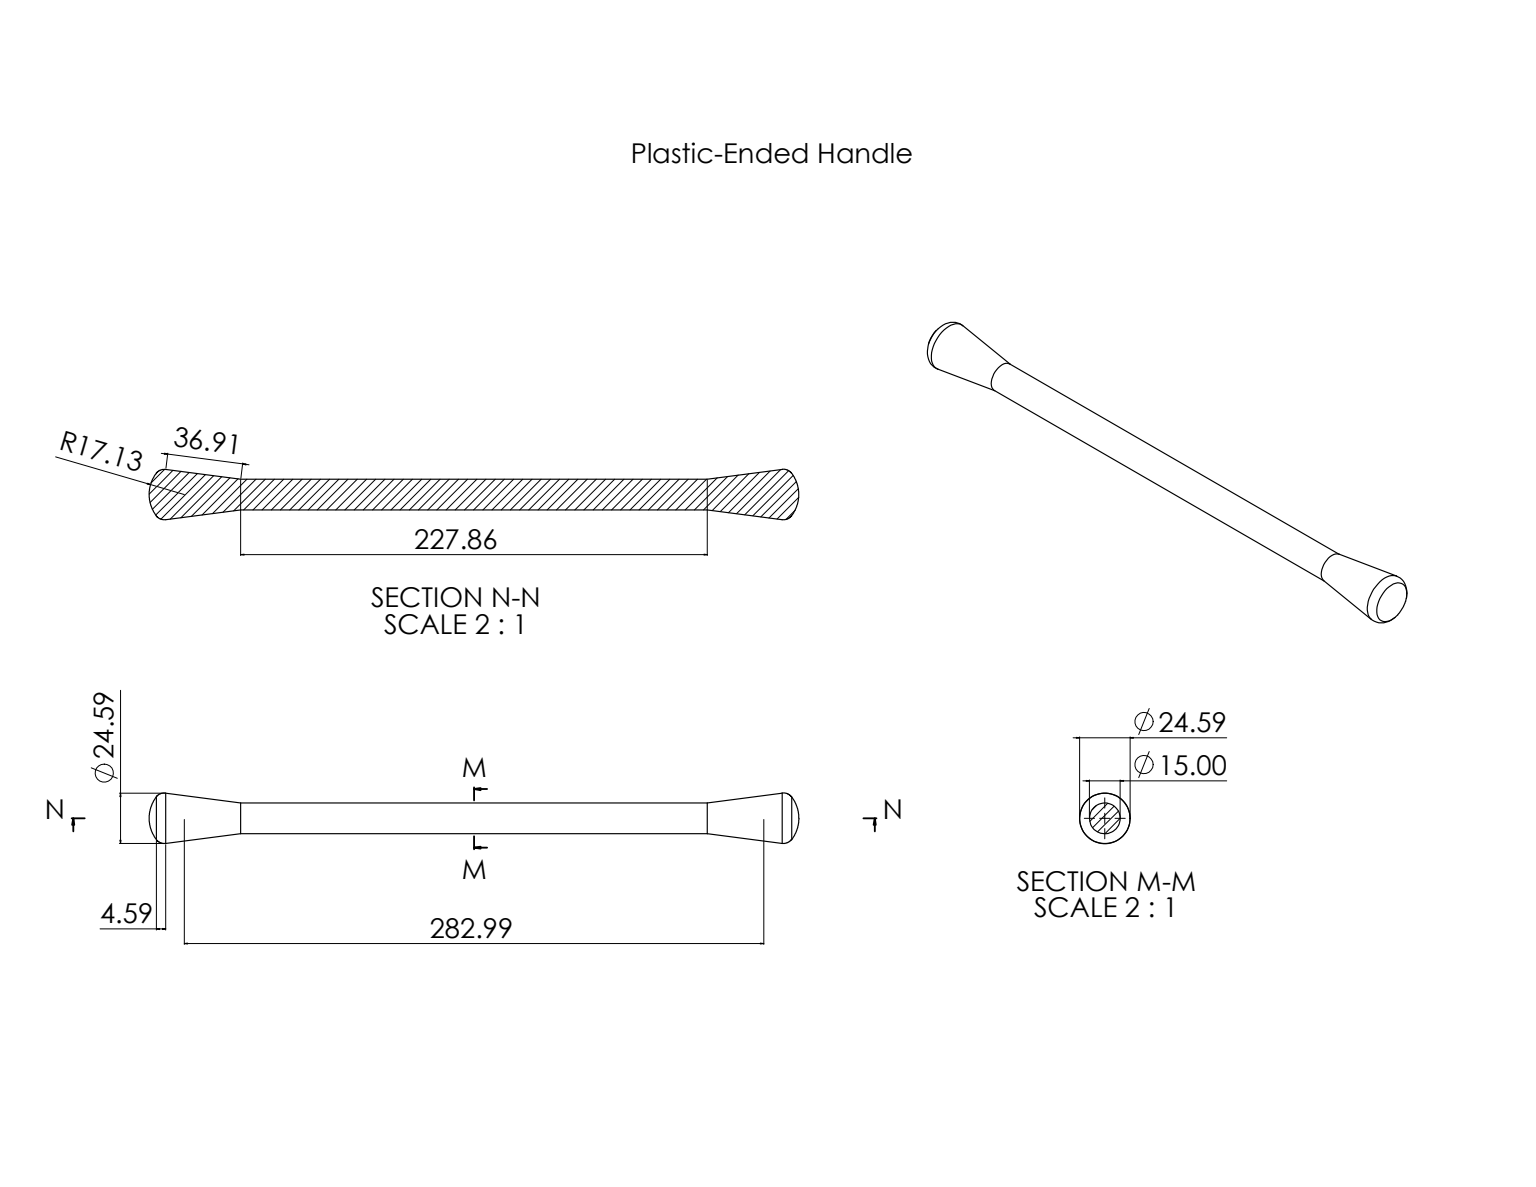
ISO-10303-21;
HEADER;
FILE_DESCRIPTION (('STEP AP214'),
    '1' );
FILE_NAME ('Plastic-Ended Handle.step',
    '2026-10-21T18:33:49',
    ( '' ),
    ( '' ),
    'SwSTEP 2.0',
    'SolidWorks 2025',
    '' );
FILE_SCHEMA (( 'AUTOMOTIVE_DESIGN' ));
ENDSEC;

DATA;
#11=AXIS2_PLACEMENT_3D ( 'NONE', #13563, #6445, #16272 ) ;
#14=ORIENTED_EDGE ( 'NONE', *, *, #12006, .F. ) ;
#41=LINE ( 'NONE', #15673, #2725 ) ;
#85=( NAMED_UNIT ( * ) SI_UNIT ( $, .STERADIAN. ) SOLID_ANGLE_UNIT ( ) );
#126=ADVANCED_FACE ( 'NONE', ( #11640 ), #16856, .T. ) ;
#152=MANIFOLD_SOLID_BREP ( 'Revolve1', #15042 ) ;
#157=CIRCLE ( 'NONE', #3134, 10.38004356723770627 ) ;
#223=DIRECTION ( 'NONE',  ( 0.000000000000000000, -0.000000000000000000, 1.000000000000000000 ) ) ;
#307=CIRCLE ( 'NONE', #13165, 4.962965561209093046 ) ;
#345=ORIENTED_EDGE ( 'NONE', *, *, #13737, .F. ) ;
#374=CARTESIAN_POINT ( 'NONE',  ( -212.2032458117903104, 84.22855780814606419, 52.11995643276230794 ) ) ;
#389=DIRECTION ( 'NONE',  ( 0.000000000000000000, 0.000000000000000000, 1.000000000000000000 ) ) ;
#392=ORIENTED_EDGE ( 'NONE', *, *, #13744, .T. ) ;
#655=AXIS2_PLACEMENT_3D ( 'NONE', #13524, #709, #7704 ) ;
#658=ORIENTED_EDGE ( 'NONE', *, *, #15578, .F. ) ;
#681=CARTESIAN_POINT ( 'NONE',  ( -208.2552686774341737, 84.22855780814606419, 55.12736457073573604 ) ) ;
#709=DIRECTION ( 'NONE',  ( 0.000000000000000000, -0.000000000000000000, -1.000000000000000000 ) ) ;
#801=LINE ( 'NONE', #2012, #10914 ) ;
#819=DIRECTION ( 'NONE',  ( 0.000000000000000000, 0.000000000000000000, -1.000000000000000000 ) ) ;
#822=EDGE_CURVE ( 'NONE', #1101, #833, #157, .T. ) ;
#833=VERTEX_POINT ( 'NONE', #374 ) ;
#864=VERTEX_POINT ( 'NONE', #11793 ) ;
#905=FACE_OUTER_BOUND ( 'NONE', #13588, .T. ) ;
#932=CARTESIAN_POINT ( 'NONE',  ( -171.0109138863553824, 84.22855780814606419, 55.00000000000000711 ) ) ;
#942=DIRECTION ( 'NONE',  ( 1.000000000000000000, -0.000000000000000000, -0.000000000000000000 ) ) ;
#992=DIRECTION ( 'NONE',  ( 0.000000000000000000, 0.000000000000000000, 1.000000000000000000 ) ) ;
#998=ORIENTED_EDGE ( 'NONE', *, *, #15679, .F. ) ;
#1033=DIRECTION ( 'NONE',  ( -0.9915318908039647550, 1.590368294782254281E-17, -0.1298634264091108326 ) ) ;
#1101=VERTEX_POINT ( 'NONE', #4112 ) ;
#1111=FACE_OUTER_BOUND ( 'NONE', #17441, .T. ) ;
#1270=ORIENTED_EDGE ( 'NONE', *, *, #2418, .T. ) ;
#1305=FACE_OUTER_BOUND ( 'NONE', #5820, .T. ) ;
#1431=EDGE_LOOP ( 'NONE', ( #9618, #16149, #15476, #8955 ) ) ;
#1443=ORIENTED_EDGE ( 'NONE', *, *, #5918, .F. ) ;
#1466=CARTESIAN_POINT ( 'NONE',  ( 93.45071565215914688, 84.22855780814606419, 62.50000000000001421 ) ) ;
#1568=ORIENTED_EDGE ( 'NONE', *, *, #6498, .F. ) ;
#1660=FACE_OUTER_BOUND ( 'NONE', #4429, .T. ) ;
#1677=SHAPE_REPRESENTATION ( 'Plastic-Ended Handle', ( #16217 ), #12057 ) ;
#1703=CARTESIAN_POINT ( 'NONE',  ( -212.2032458117903104, 84.22855780814606419, 72.88004356723772048 ) ) ;
#1752=CARTESIAN_POINT ( 'NONE',  ( 93.45071565215914688, 84.22855780814606419, 74.79357405616491405 ) ) ;
#1784=DIRECTION ( 'NONE',  ( -1.000000000000000000, -0.000000000000000000, -0.000000000000000000 ) ) ;
#1810=ADVANCED_FACE ( 'NONE', ( #905 ), #6119, .T. ) ;
#1833=AXIS2_PLACEMENT_3D ( 'NONE', #11522, #4305, #10972 ) ;
#1834=ADVANCED_FACE ( 'NONE', ( #1111 ), #9012, .T. ) ;
#1908=VERTEX_POINT ( 'NONE', #9897 ) ;
#2012=CARTESIAN_POINT ( 'NONE',  ( 97.91997734382704266, 84.22855780814606419, 70.00000000000001421 ) ) ;
#2048=EDGE_CURVE ( 'NONE', #833, #4354, #17752, .T. ) ;
#2060=FACE_OUTER_BOUND ( 'NONE', #8644, .T. ) ;
#2093=( NAMED_UNIT ( * ) SI_UNIT ( $, .STERADIAN. ) SOLID_ANGLE_UNIT ( ) );
#2118=LINE ( 'NONE', #15207, #8794 ) ;
#2381=CIRCLE ( 'NONE', #12873, 17.12963335357822814 ) ;
#2418=EDGE_CURVE ( 'NONE', #10909, #17887, #10092, .T. ) ;
#2423=LINE ( 'NONE', #932, #15542 ) ;
#2440=AXIS2_PLACEMENT_3D ( 'NONE', #5540, #18168, #13966 ) ;
#2474=CIRCLE ( 'NONE', #3078, 10.38004356723770627 ) ;
#2503=APPLICATION_CONTEXT ( 'automotive_design' ) ;
#2540=MECHANICAL_DESIGN_GEOMETRIC_PRESENTATION_REPRESENTATION('',(#6710),#15684);
#2587=CARTESIAN_POINT ( 'NONE',  ( 97.91997734382704266, 84.22855780814606419, 62.50000000000001421 ) ) ;
#2663=ADVANCED_FACE ( 'NONE', ( #6795 ), #13556, .T. ) ;
#2674=DIRECTION ( 'NONE',  ( 1.000000000000000000, -0.000000000000000000, -0.000000000000000000 ) ) ;
#2679=PRODUCT ( 'Plastic-Ended Handle', 'Plastic-Ended Handle', '', ( #6865 ) ) ;
#2725=VECTOR ( 'NONE', #8469, 1000.000000000000000 ) ;
#2771=CARTESIAN_POINT ( 'NONE',  ( 84.41679105416972106, 84.22855780814606419, 62.50000000000001421 ) ) ;
#2872=AXIS2_PLACEMENT_3D ( 'NONE', #13058, #223, #8747 ) ;
#2969=CARTESIAN_POINT ( 'NONE',  ( 93.45071565215914688, 84.22855780814606419, 62.50000000000001421 ) ) ;
#3004=DIRECTION ( 'NONE',  ( 1.000000000000000000, -0.000000000000000000, -0.000000000000000000 ) ) ;
#3050=VERTEX_POINT ( 'NONE', #1703 ) ;
#3078=AXIS2_PLACEMENT_3D ( 'NONE', #6362, #9279, #12180 ) ;
#3122=AXIS2_PLACEMENT_3D ( 'NONE', #7521, #10240, #8854 ) ;
#3134=AXIS2_PLACEMENT_3D ( 'NONE', #4485, #3004, #15904 ) ;
#3167=VERTEX_POINT ( 'NONE', #6171 ) ;
#3255=ORIENTED_EDGE ( 'NONE', *, *, #15679, .T. ) ;
#3357=DIRECTION ( 'NONE',  ( -1.000000000000000000, 0.000000000000000000, 0.000000000000000000 ) ) ;
#3455=ORIENTED_EDGE ( 'NONE', *, *, #9148, .T. ) ;
#3495=DIRECTION ( 'NONE',  ( 1.000000000000000000, -0.000000000000000000, -0.000000000000000000 ) ) ;
#3565=DIRECTION ( 'NONE',  ( 0.000000000000000000, 1.000000000000000000, 0.000000000000000000 ) ) ;
#3837=AXIS2_PLACEMENT_3D ( 'NONE', #3931, #5242, #9543 ) ;
#3850=DIRECTION ( 'NONE',  ( 0.000000000000000000, 0.000000000000000000, -1.000000000000000000 ) ) ;
#3862=( NAMED_UNIT ( * ) PLANE_ANGLE_UNIT ( ) SI_UNIT ( $, .RADIAN. ) );
#3931=CARTESIAN_POINT ( 'NONE',  ( 56.85086857400936822, 84.22855780814606419, 62.50000000000001421 ) ) ;
#3950=DIRECTION ( 'NONE',  ( 0.000000000000000000, 1.000000000000000000, 0.000000000000000000 ) ) ;
#4112=CARTESIAN_POINT ( 'NONE',  ( -212.2032458117903104, 73.84851424090838634, 62.50000000000001421 ) ) ;
#4252=DIRECTION ( 'NONE',  ( 0.000000000000000000, 0.000000000000000000, -1.000000000000000000 ) ) ;
#4305=DIRECTION ( 'NONE',  ( 1.000000000000000000, -0.000000000000000000, -0.000000000000000000 ) ) ;
#4354=VERTEX_POINT ( 'NONE', #16482 ) ;
#4429=EDGE_LOOP ( 'NONE', ( #18514, #18372, #3255, #18470 ) ) ;
#4449=EDGE_CURVE ( 'NONE', #864, #1101, #2381, .T. ) ;
#4485=CARTESIAN_POINT ( 'NONE',  ( -212.2032458117903104, 84.22855780814606419, 62.50000000000001421 ) ) ;
#4558=DIRECTION ( 'NONE',  ( 0.000000000000000000, 0.000000000000000000, -1.000000000000000000 ) ) ;
#4603=EDGE_CURVE ( 'NONE', #1908, #12880, #7466, .T. ) ;
#4635=AXIS2_PLACEMENT_3D ( 'NONE', #7678, #1784, #389 ) ;
#4769=ORIENTED_EDGE ( 'NONE', *, *, #822, .T. ) ;
#4877=DIRECTION ( 'NONE',  ( -0.9915318908039647550, 0.000000000000000000, 0.1298634264091108326 ) ) ;
#4894=CARTESIAN_POINT ( 'NONE',  ( -208.2552686774341737, 84.22855780814606419, 62.50000000000001421 ) ) ;
#4987=CARTESIAN_POINT ( 'NONE',  ( -212.2032458117903104, 84.22855780814606419, 62.50000000000001421 ) ) ;
#5020=EDGE_CURVE ( 'NONE', #17887, #12880, #307, .T. ) ;
#5087=ORIENTED_EDGE ( 'NONE', *, *, #6881, .T. ) ;
#5184=ORIENTED_EDGE ( 'NONE', *, *, #4449, .F. ) ;
#5223=ORIENTED_EDGE ( 'NONE', *, *, #8129, .T. ) ;
#5241=CIRCLE ( 'NONE', #18404, 10.38004356723770627 ) ;
#5242=DIRECTION ( 'NONE',  ( 1.000000000000000000, -0.000000000000000000, -0.000000000000000000 ) ) ;
#5280=EDGE_CURVE ( 'NONE', #14482, #14175, #17268, .T. ) ;
#5289=DIRECTION ( 'NONE',  ( 1.000000000000000000, 0.000000000000000000, 0.000000000000000000 ) ) ;
#5337=VERTEX_POINT ( 'NONE', #6377 ) ;
#5425=VERTEX_POINT ( 'NONE', #12004 ) ;
#5500=DIRECTION ( 'NONE',  ( 1.000000000000000000, -0.000000000000000000, -0.000000000000000000 ) ) ;
#5540=CARTESIAN_POINT ( 'NONE',  ( -207.6107609645051753, 84.22855780814606419, 62.50000000000001421 ) ) ;
#5575=ORIENTED_EDGE ( 'NONE', *, *, #7982, .T. ) ;
#5647=DIRECTION ( 'NONE',  ( 1.000000000000000000, -0.000000000000000000, -0.000000000000000000 ) ) ;
#5720=DIRECTION ( 'NONE',  ( 0.000000000000000000, 1.224646799147353207E-16, 1.000000000000000000 ) ) ;
#5750=CIRCLE ( 'NONE', #6638, 7.500000000000007105 ) ;
#5781=CARTESIAN_POINT ( 'NONE',  ( 0.000000000000000000, 0.000000000000000000, 0.000000000000000000 ) ) ;
#5800=CIRCLE ( 'NONE', #7899, 10.38004356723770627 ) ;
#5820=EDGE_LOOP ( 'NONE', ( #10610, #14671, #3455, #345 ) ) ;
#5883=CARTESIAN_POINT ( 'NONE',  ( 98.04320049944426785, 84.22855780814606419, 62.50000000000001421 ) ) ;
#5898=ADVANCED_BREP_SHAPE_REPRESENTATION ( '', ( #152, #16217 ), #12057 ) ;
#5918=EDGE_CURVE ( 'NONE', #10909, #5337, #12211, .T. ) ;
#6005=ORIENTED_EDGE ( 'NONE', *, *, #9042, .T. ) ;
#6011=CIRCLE ( 'NONE', #2440, 12.29357405616490695 ) ;
#6037=DIRECTION ( 'NONE',  ( 0.000000000000000000, 0.000000000000000000, 1.000000000000000000 ) ) ;
#6117=EDGE_CURVE ( 'NONE', #12880, #3167, #8386, .T. ) ;
#6119=CONICAL_SURFACE ( 'NONE', #16585, 12.29357405616490695, 0.1302312384721128480 ) ;
#6171=CARTESIAN_POINT ( 'NONE',  ( 98.04320049944426785, 94.60860137538374204, 62.50000000000001421 ) ) ;
#6215=( LENGTH_UNIT ( ) NAMED_UNIT ( * ) SI_UNIT ( .MILLI., .METRE. ) );
#6362=CARTESIAN_POINT ( 'NONE',  ( -212.2032458117903104, 84.22855780814606419, 62.50000000000001421 ) ) ;
#6377=CARTESIAN_POINT ( 'NONE',  ( 56.85086857400936822, 84.22855780814606419, 70.00000000000001421 ) ) ;
#6445=DIRECTION ( 'NONE',  ( 0.000000000000000000, 1.000000000000000000, -1.224646799147353207E-16 ) ) ;
#6498=EDGE_CURVE ( 'NONE', #5337, #11425, #41, .T. ) ;
#6559=DIRECTION ( 'NONE',  ( -0.000000000000000000, -1.000000000000000000, -0.000000000000000000 ) ) ;
#6579=DIRECTION ( 'NONE',  ( 1.000000000000000000, -0.000000000000000000, -0.000000000000000000 ) ) ;
#6620=ORIENTED_EDGE ( 'NONE', *, *, #5280, .T. ) ;
#6638=AXIS2_PLACEMENT_3D ( 'NONE', #15753, #11720, #15836 ) ;
#6652=UNCERTAINTY_MEASURE_WITH_UNIT (LENGTH_MEASURE( 1.000000000000000082E-05 ), #6215, 'distance_accuracy_value', 'NONE');
#6676=ORIENTED_EDGE ( 'NONE', *, *, #12311, .F. ) ;
#6692=DIRECTION ( 'NONE',  ( 0.000000000000000000, 0.000000000000000000, -1.000000000000000000 ) ) ;
#6710=STYLED_ITEM('',(#18545),#152);
#6795=FACE_OUTER_BOUND ( 'NONE', #10659, .T. ) ;
#6865=PRODUCT_CONTEXT ( 'NONE', #2503, 'mechanical' ) ;
#6881=EDGE_CURVE ( 'NONE', #11425, #17887, #14110, .T. ) ;
#6921=AXIS2_PLACEMENT_3D ( 'NONE', #18476, #5647, #4252 ) ;
#7039=FACE_OUTER_BOUND ( 'NONE', #11821, .T. ) ;
#7136=VERTEX_POINT ( 'NONE', #14683 ) ;
#7191=SHAPE_REPRESENTATION_RELATIONSHIP ( 'NONE' , 'NONE' ,  #1677, #5898 ) ;
#7208=CARTESIAN_POINT ( 'NONE',  ( 94.09522336508815954, 84.22855780814606419, 62.50000000000001421 ) ) ;
#7369=DIRECTION ( 'NONE',  ( 0.000000000000000000, -0.000000000000000000, -1.000000000000000000 ) ) ;
#7370=CARTESIAN_POINT ( 'NONE',  ( -171.0109138863553824, 84.22855780814606419, 62.50000000000001421 ) ) ;
#7387=DIRECTION ( 'NONE',  ( 0.000000000000000000, 0.000000000000000000, -1.000000000000000000 ) ) ;
#7420=EDGE_LOOP ( 'NONE', ( #17630, #16514, #6005, #16324 ) ) ;
#7466=CIRCLE ( 'NONE', #17907, 10.38004356723770627 ) ;
#7520=AXIS2_PLACEMENT_3D ( 'NONE', #13096, #9923, #11596 ) ;
#7521=CARTESIAN_POINT ( 'NONE',  ( -208.2552686774341737, 84.22855780814606419, 62.50000000000001421 ) ) ;
#7546=DIRECTION ( 'NONE',  ( 0.9915318908039647550, 0.000000000000000000, -0.1298634264091108326 ) ) ;
#7566=ADVANCED_FACE ( 'NONE', ( #7711 ), #14905, .T. ) ;
#7654=CARTESIAN_POINT ( 'NONE',  ( 94.09522336508815954, 84.22855780814606419, 55.12736457073573604 ) ) ;
#7662=ADVANCED_FACE ( 'NONE', ( #10699 ), #10517, .T. ) ;
#7678=CARTESIAN_POINT ( 'NONE',  ( 97.91997734382704266, 84.22855780814606419, 62.50000000000001421 ) ) ;
#7681=ORIENTED_EDGE ( 'NONE', *, *, #12311, .T. ) ;
#7704=DIRECTION ( 'NONE',  ( 0.000000000000000000, -1.000000000000000000, 0.000000000000000000 ) ) ;
#7711=FACE_OUTER_BOUND ( 'NONE', #1431, .T. ) ;
#7771=ORIENTED_EDGE ( 'NONE', *, *, #9729, .F. ) ;
#7776=CARTESIAN_POINT ( 'NONE',  ( 93.45071565215914688, 84.22855780814606419, 50.20642594383511437 ) ) ;
#7858=DIRECTION ( 'NONE',  ( 0.000000000000000000, 0.000000000000000000, -1.000000000000000000 ) ) ;
#7899=AXIS2_PLACEMENT_3D ( 'NONE', #4987, #6579, #10620 ) ;
#7982=EDGE_CURVE ( 'NONE', #5337, #10909, #5750, .T. ) ;
#8040=AXIS2_PLACEMENT_3D ( 'NONE', #7370, #13083, #10353 ) ;
#8054=DIRECTION ( 'NONE',  ( 1.000000000000000000, -0.000000000000000000, -0.000000000000000000 ) ) ;
#8064=CIRCLE ( 'NONE', #11, 4.962965561209093046 ) ;
#8129=EDGE_CURVE ( 'NONE', #10654, #3050, #2474, .T. ) ;
#8264=ORIENTED_EDGE ( 'NONE', *, *, #11575, .T. ) ;
#8310=ORIENTED_EDGE ( 'NONE', *, *, #6117, .F. ) ;
#8336=PRODUCT_DEFINITION_CONTEXT ( 'detailed design', #8853, 'design' ) ;
#8355=PRODUCT_DEFINITION_SHAPE ( 'NONE', 'NONE',  #15399 ) ;
#8386=CIRCLE ( 'NONE', #14361, 10.38004356723770627 ) ;
#8469=DIRECTION ( 'NONE',  ( 0.9915318908039647550, 1.590368294782254281E-17, 0.1298634264091108326 ) ) ;
#8472=EDGE_LOOP ( 'NONE', ( #5223, #16778, #998, #9687, #11073 ) ) ;
#8490=CARTESIAN_POINT ( 'NONE',  ( 56.85086857400936822, 84.22855780814606419, 55.00000000000000711 ) ) ;
#8493=PRODUCT_DEFINITION_FORMATION_WITH_SPECIFIED_SOURCE ( 'ANY', '', #2679, .NOT_KNOWN. ) ;
#8644=EDGE_LOOP ( 'NONE', ( #1443, #8264, #6620, #9226 ) ) ;
#8705=CARTESIAN_POINT ( 'NONE',  ( -171.0109138863553824, 84.22855780814606419, 70.00000000000001421 ) ) ;
#8747=DIRECTION ( 'NONE',  ( 0.000000000000000000, 1.000000000000000000, 0.000000000000000000 ) ) ;
#8794=VECTOR ( 'NONE', #15121, 1000.000000000000000 ) ;
#8853=APPLICATION_CONTEXT ( 'automotive_design' ) ;
#8854=DIRECTION ( 'NONE',  ( 0.000000000000000000, 0.000000000000000000, -1.000000000000000000 ) ) ;
#8904=CYLINDRICAL_SURFACE ( 'NONE', #4635, 7.500000000000007105 ) ;
#8953=EDGE_CURVE ( 'NONE', #833, #10654, #12905, .T. ) ;
#8955=ORIENTED_EDGE ( 'NONE', *, *, #13737, .T. ) ;
#8961=DIRECTION ( 'NONE',  ( 1.000000000000000000, 0.000000000000000000, 0.000000000000000000 ) ) ;
#8974=AXIS2_PLACEMENT_3D ( 'NONE', #10668, #16355, #9447 ) ;
#9012=SPHERICAL_SURFACE ( 'NONE', #2872, 17.12963335357822103 ) ;
#9042=EDGE_CURVE ( 'NONE', #14175, #7136, #16471, .T. ) ;
#9118=ORIENTED_EDGE ( 'NONE', *, *, #2418, .F. ) ;
#9148=EDGE_CURVE ( 'NONE', #3167, #5425, #17661, .T. ) ;
#9164=EDGE_CURVE ( 'NONE', #7136, #4354, #6011, .T. ) ;
#9226=ORIENTED_EDGE ( 'NONE', *, *, #13607, .F. ) ;
#9279=DIRECTION ( 'NONE',  ( 1.000000000000000000, -0.000000000000000000, -0.000000000000000000 ) ) ;
#9299=DIRECTION ( 'NONE',  ( 0.000000000000000000, 0.000000000000000000, -1.000000000000000000 ) ) ;
#9338=AXIS2_PLACEMENT_3D ( 'NONE', #4894, #3495, #9299 ) ;
#9360=CARTESIAN_POINT ( 'NONE',  ( 98.04320049944426785, 84.22855780814606419, 62.50000000000001421 ) ) ;
#9447=DIRECTION ( 'NONE',  ( 0.000000000000000000, 0.000000000000000000, -1.000000000000000000 ) ) ;
#9468=DIRECTION ( 'NONE',  ( 0.000000000000000000, 0.000000000000000000, -1.000000000000000000 ) ) ;
#9482=DIRECTION ( 'NONE',  ( 0.000000000000000000, 0.000000000000000000, 1.000000000000000000 ) ) ;
#9541=ORIENTED_EDGE ( 'NONE', *, *, #822, .F. ) ;
#9543=DIRECTION ( 'NONE',  ( 0.000000000000000000, 0.000000000000000000, -1.000000000000000000 ) ) ;
#9585=FACE_OUTER_BOUND ( 'NONE', #12427, .T. ) ;
#9618=ORIENTED_EDGE ( 'NONE', *, *, #9148, .F. ) ;
#9687=ORIENTED_EDGE ( 'NONE', *, *, #2048, .F. ) ;
#9729=EDGE_CURVE ( 'NONE', #3050, #7136, #13223, .T. ) ;
#9784=DIRECTION ( 'NONE',  ( 0.000000000000000000, 0.000000000000000000, 1.000000000000000000 ) ) ;
#9847=DIRECTION ( 'NONE',  ( 0.000000000000000000, -0.000000000000000000, 1.000000000000000000 ) ) ;
#9875=DIRECTION ( 'NONE',  ( -1.000000000000000000, -0.000000000000000000, -0.000000000000000000 ) ) ;
#9897=CARTESIAN_POINT ( 'NONE',  ( 98.04320049944426785, 73.84851424090838634, 62.50000000000001421 ) ) ;
#9923=DIRECTION ( 'NONE',  ( 0.000000000000000000, 1.000000000000000000, -1.224646799147353207E-16 ) ) ;
#10092=LINE ( 'NONE', #11668, #12671 ) ;
#10108=DIRECTION ( 'NONE',  ( 0.000000000000000000, 0.000000000000000000, -1.000000000000000000 ) ) ;
#10240=DIRECTION ( 'NONE',  ( 1.000000000000000000, -0.000000000000000000, -0.000000000000000000 ) ) ;
#10259=DIRECTION ( 'NONE',  ( 1.000000000000000000, -0.000000000000000000, -0.000000000000000000 ) ) ;
#10353=DIRECTION ( 'NONE',  ( 0.000000000000000000, 0.000000000000000000, 1.000000000000000000 ) ) ;
#10417=ADVANCED_FACE ( 'NONE', ( #18174 ), #16755, .T. ) ;
#10517=TOROIDAL_SURFACE ( 'NONE', #9338, 7.372635429264279061, 4.962965561209096599 ) ;
#10610=ORIENTED_EDGE ( 'NONE', *, *, #4603, .T. ) ;
#10620=DIRECTION ( 'NONE',  ( 0.000000000000000000, 0.000000000000000000, -1.000000000000000000 ) ) ;
#10654=VERTEX_POINT ( 'NONE', #12258 ) ;
#10659=EDGE_LOOP ( 'NONE', ( #14138, #18278, #17509, #8310, #16101 ) ) ;
#10668=CARTESIAN_POINT ( 'NONE',  ( -207.6107609645051753, 84.22855780814606419, 62.50000000000001421 ) ) ;
#10699=FACE_OUTER_BOUND ( 'NONE', #8472, .T. ) ;
#10768=AXIS2_PLACEMENT_3D ( 'NONE', #7208, #17121, #10108 ) ;
#10909=VERTEX_POINT ( 'NONE', #8490 ) ;
#10914=VECTOR ( 'NONE', #15109, 1000.000000000000000 ) ;
#10971=CARTESIAN_POINT ( 'NONE',  ( 93.45071565215914688, 84.22855780814606419, 62.50000000000001421 ) ) ;
#10972=DIRECTION ( 'NONE',  ( 0.000000000000000000, 0.000000000000000000, -1.000000000000000000 ) ) ;
#11019=CARTESIAN_POINT ( 'NONE',  ( 93.45071565215914688, 84.22855780814606419, 62.50000000000001421 ) ) ;
#11073=ORIENTED_EDGE ( 'NONE', *, *, #8953, .T. ) ;
#11094=CARTESIAN_POINT ( 'NONE',  ( -171.0109138863553824, 84.22855780814606419, 62.50000000000001421 ) ) ;
#11102=VECTOR ( 'NONE', #4877, 1000.000000000000000 ) ;
#11222=CIRCLE ( 'NONE', #15090, 17.12963335357822814 ) ;
#11223=AXIS2_PLACEMENT_3D ( 'NONE', #14592, #11799, #3357 ) ;
#11235=AXIS2_PLACEMENT_3D ( 'NONE', #11094, #2674, #6692 ) ;
#11396=DIRECTION ( 'NONE',  ( 1.000000000000000000, -0.000000000000000000, -0.000000000000000000 ) ) ;
#11425=VERTEX_POINT ( 'NONE', #1752 ) ;
#11498=DIRECTION ( 'NONE',  ( 0.000000000000000000, -1.000000000000000000, 0.000000000000000000 ) ) ;
#11502=AXIS2_PLACEMENT_3D ( 'NONE', #1466, #11396, #12892 ) ;
#11522=CARTESIAN_POINT ( 'NONE',  ( 98.04320049944426785, 84.22855780814606419, 62.50000000000001421 ) ) ;
#11544=DIRECTION ( 'NONE',  ( 0.000000000000000000, -1.000000000000000000, 0.000000000000000000 ) ) ;
#11575=EDGE_CURVE ( 'NONE', #10909, #14482, #2118, .T. ) ;
#11582=CARTESIAN_POINT ( 'NONE',  ( 84.41679105416972106, 84.22855780814606419, 62.50000000000001421 ) ) ;
#11596=DIRECTION ( 'NONE',  ( 0.000000000000000000, 0.000000000000000000, 1.000000000000000000 ) ) ;
#11640=FACE_OUTER_BOUND ( 'NONE', #14929, .T. ) ;
#11668=CARTESIAN_POINT ( 'NONE',  ( 93.45071565215914688, 84.22855780814606419, 50.20642594383510726 ) ) ;
#11716=ORIENTED_EDGE ( 'NONE', *, *, #11575, .F. ) ;
#11720=DIRECTION ( 'NONE',  ( 1.000000000000000000, -0.000000000000000000, -0.000000000000000000 ) ) ;
#11755=SPHERICAL_SURFACE ( 'NONE', #16567, 17.12963335357822103 ) ;
#11780=ADVANCED_FACE ( 'NONE', ( #15701 ), #13578, .T. ) ;
#11793=CARTESIAN_POINT ( 'NONE',  ( -215.7064697200939634, 84.22855780814606419, 62.50000000000001421 ) ) ;
#11799=DIRECTION ( 'NONE',  ( 0.000000000000000000, 0.000000000000000000, -1.000000000000000000 ) ) ;
#11821=EDGE_LOOP ( 'NONE', ( #658, #5087, #17884, #12096, #14504 ) ) ;
#11829=EDGE_LOOP ( 'NONE', ( #5184, #7681, #16456, #9541 ) ) ;
#11992=CARTESIAN_POINT ( 'NONE',  ( -171.0109138863553824, 84.22855780814606419, 70.00000000000001421 ) ) ;
#12004=CARTESIAN_POINT ( 'NONE',  ( 101.5464244077479492, 84.22855780814606419, 62.50000000000001421 ) ) ;
#12006=EDGE_CURVE ( 'NONE', #3050, #1101, #5800, .T. ) ;
#12016=ADVANCED_FACE ( 'NONE', ( #16494 ), #14768, .T. ) ;
#12057=( GEOMETRIC_REPRESENTATION_CONTEXT ( 3 ) GLOBAL_UNCERTAINTY_ASSIGNED_CONTEXT ( ( #6652 ) ) GLOBAL_UNIT_ASSIGNED_CONTEXT ( ( #6215, #12140, #85 ) ) REPRESENTATION_CONTEXT ( 'NONE', 'WORKASPACE' ) );
#12095=DIRECTION ( 'NONE',  ( -0.000000000000000000, -1.224646799147353207E-16, -1.000000000000000000 ) ) ;
#12096=ORIENTED_EDGE ( 'NONE', *, *, #4603, .F. ) ;
#12114=( LENGTH_UNIT ( ) NAMED_UNIT ( * ) SI_UNIT ( .MILLI., .METRE. ) );
#12140=( NAMED_UNIT ( * ) PLANE_ANGLE_UNIT ( ) SI_UNIT ( $, .RADIAN. ) );
#12180=DIRECTION ( 'NONE',  ( 0.000000000000000000, 0.000000000000000000, -1.000000000000000000 ) ) ;
#12211=CIRCLE ( 'NONE', #3837, 7.500000000000007105 ) ;
#12258=CARTESIAN_POINT ( 'NONE',  ( -212.2032458117903104, 94.60860137538374204, 62.50000000000001421 ) ) ;
#12273=CIRCLE ( 'NONE', #12852, 12.29357405616490695 ) ;
#12303=CARTESIAN_POINT ( 'NONE',  ( -171.0109138863553824, 84.22855780814606419, 62.50000000000001421 ) ) ;
#12311=EDGE_CURVE ( 'NONE', #864, #10654, #17766, .T. ) ;
#12419=CIRCLE ( 'NONE', #11235, 7.500000000000007105 ) ;
#12427=EDGE_LOOP ( 'NONE', ( #11716, #15732, #18422, #392 ) ) ;
#12507=CYLINDRICAL_SURFACE ( 'NONE', #13526, 7.500000000000007105 ) ;
#12515=DIRECTION ( 'NONE',  ( 1.000000000000000000, -0.000000000000000000, -0.000000000000000000 ) ) ;
#12612=ORIENTED_EDGE ( 'NONE', *, *, #6498, .T. ) ;
#12631=EDGE_CURVE ( 'NONE', #18012, #1908, #5241, .T. ) ;
#12671=VECTOR ( 'NONE', #7546, 1000.000000000000000 ) ;
#12852=AXIS2_PLACEMENT_3D ( 'NONE', #2969, #10259, #14646 ) ;
#12873=AXIS2_PLACEMENT_3D ( 'NONE', #17228, #5720, #11544 ) ;
#12880=VERTEX_POINT ( 'NONE', #14590 ) ;
#12892=DIRECTION ( 'NONE',  ( 0.000000000000000000, 0.000000000000000000, -1.000000000000000000 ) ) ;
#12905=CIRCLE ( 'NONE', #6921, 10.38004356723770627 ) ;
#12990=ORIENTED_EDGE ( 'NONE', *, *, #8129, .F. ) ;
#13058=CARTESIAN_POINT ( 'NONE',  ( -198.5768363665157494, 84.22855780814606419, 62.50000000000001421 ) ) ;
#13083=DIRECTION ( 'NONE',  ( -1.000000000000000000, 0.000000000000000000, 0.000000000000000000 ) ) ;
#13096=CARTESIAN_POINT ( 'NONE',  ( -208.2552686774341737, 84.22855780814606419, 69.87263542926429238 ) ) ;
#13165=AXIS2_PLACEMENT_3D ( 'NONE', #7654, #14666, #16061 ) ;
#13169=TOROIDAL_SURFACE ( 'NONE', #10768, 7.372635429264279061, 4.962965561209096599 ) ;
#13195=AXIS2_PLACEMENT_3D ( 'NONE', #14797, #12095, #3565 ) ;
#13223=CIRCLE ( 'NONE', #7520, 4.962965561209093046 ) ;
#13443=ADVANCED_FACE ( 'NONE', ( #1305 ), #11755, .T. ) ;
#13524=CARTESIAN_POINT ( 'NONE',  ( 84.41679105416972106, 84.22855780814606419, 62.50000000000001421 ) ) ;
#13526=AXIS2_PLACEMENT_3D ( 'NONE', #2587, #9875, #9784 ) ;
#13556=TOROIDAL_SURFACE ( 'NONE', #16220, 7.372635429264279061, 4.962965561209096599 ) ;
#13563=CARTESIAN_POINT ( 'NONE',  ( 94.09522336508815954, 84.22855780814606419, 69.87263542926429238 ) ) ;
#13578=CONICAL_SURFACE ( 'NONE', #11502, 12.29357405616490695, 0.1302312384721128480 ) ;
#13588=EDGE_LOOP ( 'NONE', ( #18200, #12612, #14764, #9118 ) ) ;
#13607=EDGE_CURVE ( 'NONE', #5337, #14175, #801, .T. ) ;
#13641=DIRECTION ( 'NONE',  ( 1.000000000000000000, -0.000000000000000000, -0.000000000000000000 ) ) ;
#13737=EDGE_CURVE ( 'NONE', #1908, #5425, #11222, .T. ) ;
#13744=EDGE_CURVE ( 'NONE', #14175, #14482, #12419, .T. ) ;
#13791=CIRCLE ( 'NONE', #1833, 10.38004356723770627 ) ;
#13809=CARTESIAN_POINT ( 'NONE',  ( 94.09522336508815954, 84.22855780814606419, 62.50000000000001421 ) ) ;
#13883=AXIS2_PLACEMENT_3D ( 'NONE', #681, #6559, #9468 ) ;
#13935=ORIENTED_EDGE ( 'NONE', *, *, #2048, .T. ) ;
#13950=ADVANCED_FACE ( 'NONE', ( #2060 ), #8904, .T. ) ;
#13966=DIRECTION ( 'NONE',  ( 0.000000000000000000, 0.000000000000000000, -1.000000000000000000 ) ) ;
#14101=DIRECTION ( 'NONE',  ( 0.000000000000000000, 0.000000000000000000, -1.000000000000000000 ) ) ;
#14110=CIRCLE ( 'NONE', #14972, 12.29357405616490695 ) ;
#14138=ORIENTED_EDGE ( 'NONE', *, *, #14604, .T. ) ;
#14158=CARTESIAN_POINT ( 'NONE',  ( -198.5768363665157494, 84.22855780814606419, 62.50000000000001421 ) ) ;
#14175=VERTEX_POINT ( 'NONE', #8705 ) ;
#14210=ADVANCED_FACE ( 'NONE', ( #7039 ), #13169, .T. ) ;
#14361=AXIS2_PLACEMENT_3D ( 'NONE', #5883, #14502, #7387 ) ;
#14373=EDGE_LOOP ( 'NONE', ( #1568, #5575, #1270, #16384 ) ) ;
#14482=VERTEX_POINT ( 'NONE', #18507 ) ;
#14502=DIRECTION ( 'NONE',  ( 1.000000000000000000, -0.000000000000000000, -0.000000000000000000 ) ) ;
#14504=ORIENTED_EDGE ( 'NONE', *, *, #12631, .F. ) ;
#14590=CARTESIAN_POINT ( 'NONE',  ( 98.04320049944426785, 84.22855780814606419, 52.11995643276230794 ) ) ;
#14592=CARTESIAN_POINT ( 'NONE',  ( -198.5768363665157494, 84.22855780814606419, 62.50000000000001421 ) ) ;
#14604=EDGE_CURVE ( 'NONE', #17887, #11425, #12273, .T. ) ;
#14646=DIRECTION ( 'NONE',  ( 0.000000000000000000, 0.000000000000000000, -1.000000000000000000 ) ) ;
#14652=CONICAL_SURFACE ( 'NONE', #8040, 7.500000000000007105, 0.1302312384721128480 ) ;
#14666=DIRECTION ( 'NONE',  ( -0.000000000000000000, -1.000000000000000000, -0.000000000000000000 ) ) ;
#14671=ORIENTED_EDGE ( 'NONE', *, *, #6117, .T. ) ;
#14683=CARTESIAN_POINT ( 'NONE',  ( -207.6107609645051753, 84.22855780814606419, 74.79357405616491405 ) ) ;
#14718=ADVANCED_FACE ( 'NONE', ( #1660 ), #14652, .T. ) ;
#14764=ORIENTED_EDGE ( 'NONE', *, *, #14604, .F. ) ;
#14768=CONICAL_SURFACE ( 'NONE', #15691, 7.500000000000007105, 0.1302312384721128480 ) ;
#14797=CARTESIAN_POINT ( 'NONE',  ( 84.41679105416972106, 84.22855780814606419, 62.50000000000001421 ) ) ;
#14905=SPHERICAL_SURFACE ( 'NONE', #655, 17.12963335357822103 ) ;
#14929=EDGE_LOOP ( 'NONE', ( #7771, #17167, #4769, #13935, #15494 ) ) ;
#14972=AXIS2_PLACEMENT_3D ( 'NONE', #10971, #8054, #3850 ) ;
#15042=CLOSED_SHELL ( 'NONE', ( #14718, #7662, #1834, #13950, #1810, #2663, #13443, #7566, #14210, #11780, #17701, #10417, #126, #12016 ) ) ;
#15090=AXIS2_PLACEMENT_3D ( 'NONE', #2771, #992, #5289 ) ;
#15109=DIRECTION ( 'NONE',  ( -1.000000000000000000, -0.000000000000000000, -0.000000000000000000 ) ) ;
#15121=DIRECTION ( 'NONE',  ( -1.000000000000000000, -0.000000000000000000, -0.000000000000000000 ) ) ;
#15175=AXIS2_PLACEMENT_3D ( 'NONE', #18328, #5500, #16913 ) ;
#15207=CARTESIAN_POINT ( 'NONE',  ( 97.91997734382704266, 84.22855780814606419, 55.00000000000001421 ) ) ;
#15399=PRODUCT_DEFINITION ( 'UNKNOWN', '', #8493, #8336 ) ;
#15476=ORIENTED_EDGE ( 'NONE', *, *, #12631, .T. ) ;
#15494=ORIENTED_EDGE ( 'NONE', *, *, #9164, .F. ) ;
#15542=VECTOR ( 'NONE', #1033, 1000.000000000000000 ) ;
#15578=EDGE_CURVE ( 'NONE', #11425, #18012, #8064, .T. ) ;
#15581=EDGE_CURVE ( 'NONE', #14482, #4354, #2423, .T. ) ;
#15643=UNCERTAINTY_MEASURE_WITH_UNIT (LENGTH_MEASURE( 1.000000000000000082E-05 ), #12114, 'distance_accuracy_value', 'NONE');
#15673=CARTESIAN_POINT ( 'NONE',  ( 93.45071565215914688, 84.22855780814606419, 74.79357405616492827 ) ) ;
#15679=EDGE_CURVE ( 'NONE', #4354, #7136, #18245, .T. ) ;
#15684=( GEOMETRIC_REPRESENTATION_CONTEXT ( 3 ) GLOBAL_UNCERTAINTY_ASSIGNED_CONTEXT ( ( #15643 ) ) GLOBAL_UNIT_ASSIGNED_CONTEXT ( ( #12114, #3862, #2093 ) ) REPRESENTATION_CONTEXT ( 'NONE', 'WORKASPACE' ) );
#15691=AXIS2_PLACEMENT_3D ( 'NONE', #12303, #16393, #9482 ) ;
#15701=FACE_OUTER_BOUND ( 'NONE', #14373, .T. ) ;
#15732=ORIENTED_EDGE ( 'NONE', *, *, #7982, .F. ) ;
#15753=CARTESIAN_POINT ( 'NONE',  ( 56.85086857400936822, 84.22855780814606419, 62.50000000000001421 ) ) ;
#15836=DIRECTION ( 'NONE',  ( 0.000000000000000000, 0.000000000000000000, -1.000000000000000000 ) ) ;
#15904=DIRECTION ( 'NONE',  ( 0.000000000000000000, 0.000000000000000000, -1.000000000000000000 ) ) ;
#16061=DIRECTION ( 'NONE',  ( 0.000000000000000000, 0.000000000000000000, -1.000000000000000000 ) ) ;
#16101=ORIENTED_EDGE ( 'NONE', *, *, #5020, .F. ) ;
#16146=DIRECTION ( 'NONE',  ( 1.000000000000000000, -0.000000000000000000, -0.000000000000000000 ) ) ;
#16149=ORIENTED_EDGE ( 'NONE', *, *, #17013, .T. ) ;
#16217=AXIS2_PLACEMENT_3D ( 'NONE', #5781, #6037, #8961 ) ;
#16220=AXIS2_PLACEMENT_3D ( 'NONE', #13809, #12515, #14101 ) ;
#16238=SHAPE_DEFINITION_REPRESENTATION ( #8355, #1677 ) ;
#16272=DIRECTION ( 'NONE',  ( 0.000000000000000000, 0.000000000000000000, 1.000000000000000000 ) ) ;
#16324=ORIENTED_EDGE ( 'NONE', *, *, #9164, .T. ) ;
#16355=DIRECTION ( 'NONE',  ( 1.000000000000000000, -0.000000000000000000, -0.000000000000000000 ) ) ;
#16384=ORIENTED_EDGE ( 'NONE', *, *, #6881, .F. ) ;
#16393=DIRECTION ( 'NONE',  ( -1.000000000000000000, 0.000000000000000000, 0.000000000000000000 ) ) ;
#16456=ORIENTED_EDGE ( 'NONE', *, *, #8953, .F. ) ;
#16471=LINE ( 'NONE', #11992, #11102 ) ;
#16482=CARTESIAN_POINT ( 'NONE',  ( -207.6107609645051753, 84.22855780814606419, 50.20642594383511437 ) ) ;
#16494=FACE_OUTER_BOUND ( 'NONE', #7420, .T. ) ;
#16514=ORIENTED_EDGE ( 'NONE', *, *, #13744, .F. ) ;
#16567=AXIS2_PLACEMENT_3D ( 'NONE', #11582, #7369, #11498 ) ;
#16585=AXIS2_PLACEMENT_3D ( 'NONE', #11019, #13641, #819 ) ;
#16755=SPHERICAL_SURFACE ( 'NONE', #17705, 17.12963335357822103 ) ;
#16778=ORIENTED_EDGE ( 'NONE', *, *, #9729, .T. ) ;
#16856=TOROIDAL_SURFACE ( 'NONE', #3122, 7.372635429264279061, 4.962965561209096599 ) ;
#16913=DIRECTION ( 'NONE',  ( 0.000000000000000000, 0.000000000000000000, -1.000000000000000000 ) ) ;
#17013=EDGE_CURVE ( 'NONE', #3167, #18012, #13791, .T. ) ;
#17121=DIRECTION ( 'NONE',  ( 1.000000000000000000, -0.000000000000000000, -0.000000000000000000 ) ) ;
#17167=ORIENTED_EDGE ( 'NONE', *, *, #12006, .T. ) ;
#17228=CARTESIAN_POINT ( 'NONE',  ( -198.5768363665157494, 84.22855780814606419, 62.50000000000001421 ) ) ;
#17268=CIRCLE ( 'NONE', #15175, 7.500000000000007105 ) ;
#17371=CARTESIAN_POINT ( 'NONE',  ( 98.04320049944426785, 84.22855780814606419, 62.50000000000001421 ) ) ;
#17441=EDGE_LOOP ( 'NONE', ( #6676, #17529, #14, #12990 ) ) ;
#17509=ORIENTED_EDGE ( 'NONE', *, *, #17013, .F. ) ;
#17529=ORIENTED_EDGE ( 'NONE', *, *, #4449, .T. ) ;
#17630=ORIENTED_EDGE ( 'NONE', *, *, #15581, .F. ) ;
#17661=CIRCLE ( 'NONE', #13195, 17.12963335357822814 ) ;
#17701=ADVANCED_FACE ( 'NONE', ( #9585 ), #12507, .T. ) ;
#17705=AXIS2_PLACEMENT_3D ( 'NONE', #14158, #9847, #3950 ) ;
#17752=CIRCLE ( 'NONE', #13883, 4.962965561209093046 ) ;
#17766=CIRCLE ( 'NONE', #11223, 17.12963335357822814 ) ;
#17884=ORIENTED_EDGE ( 'NONE', *, *, #5020, .T. ) ;
#17887=VERTEX_POINT ( 'NONE', #7776 ) ;
#17907=AXIS2_PLACEMENT_3D ( 'NONE', #9360, #942, #7858 ) ;
#18012=VERTEX_POINT ( 'NONE', #18162 ) ;
#18162=CARTESIAN_POINT ( 'NONE',  ( 98.04320049944426785, 84.22855780814606419, 72.88004356723772048 ) ) ;
#18168=DIRECTION ( 'NONE',  ( 1.000000000000000000, -0.000000000000000000, -0.000000000000000000 ) ) ;
#18174=FACE_OUTER_BOUND ( 'NONE', #11829, .T. ) ;
#18200=ORIENTED_EDGE ( 'NONE', *, *, #5918, .T. ) ;
#18245=CIRCLE ( 'NONE', #8974, 12.29357405616490695 ) ;
#18278=ORIENTED_EDGE ( 'NONE', *, *, #15578, .T. ) ;
#18328=CARTESIAN_POINT ( 'NONE',  ( -171.0109138863553824, 84.22855780814606419, 62.50000000000001421 ) ) ;
#18372=ORIENTED_EDGE ( 'NONE', *, *, #15581, .T. ) ;
#18404=AXIS2_PLACEMENT_3D ( 'NONE', #17371, #16146, #4558 ) ;
#18422=ORIENTED_EDGE ( 'NONE', *, *, #13607, .T. ) ;
#18470=ORIENTED_EDGE ( 'NONE', *, *, #9042, .F. ) ;
#18476=CARTESIAN_POINT ( 'NONE',  ( -212.2032458117903104, 84.22855780814606419, 62.50000000000001421 ) ) ;
#18507=CARTESIAN_POINT ( 'NONE',  ( -171.0109138863553824, 84.22855780814606419, 55.00000000000000711 ) ) ;
#18514=ORIENTED_EDGE ( 'NONE', *, *, #5280, .F. ) ;
#18539=COLOUR_RGB('Light Blue',0.38,0.62,0.78);
#18540=FILL_AREA_STYLE_COLOUR('',#18539);
#18541=FILL_AREA_STYLE('',(#18540));
#18542=SURFACE_STYLE_FILL_AREA(#18541);
#18543=SURFACE_SIDE_STYLE('',(#18542));
#18544=SURFACE_STYLE_USAGE(.BOTH.,#18543);
#18545=PRESENTATION_STYLE_ASSIGNMENT((#18544));
ENDSEC;
END-ISO-10303-21;
